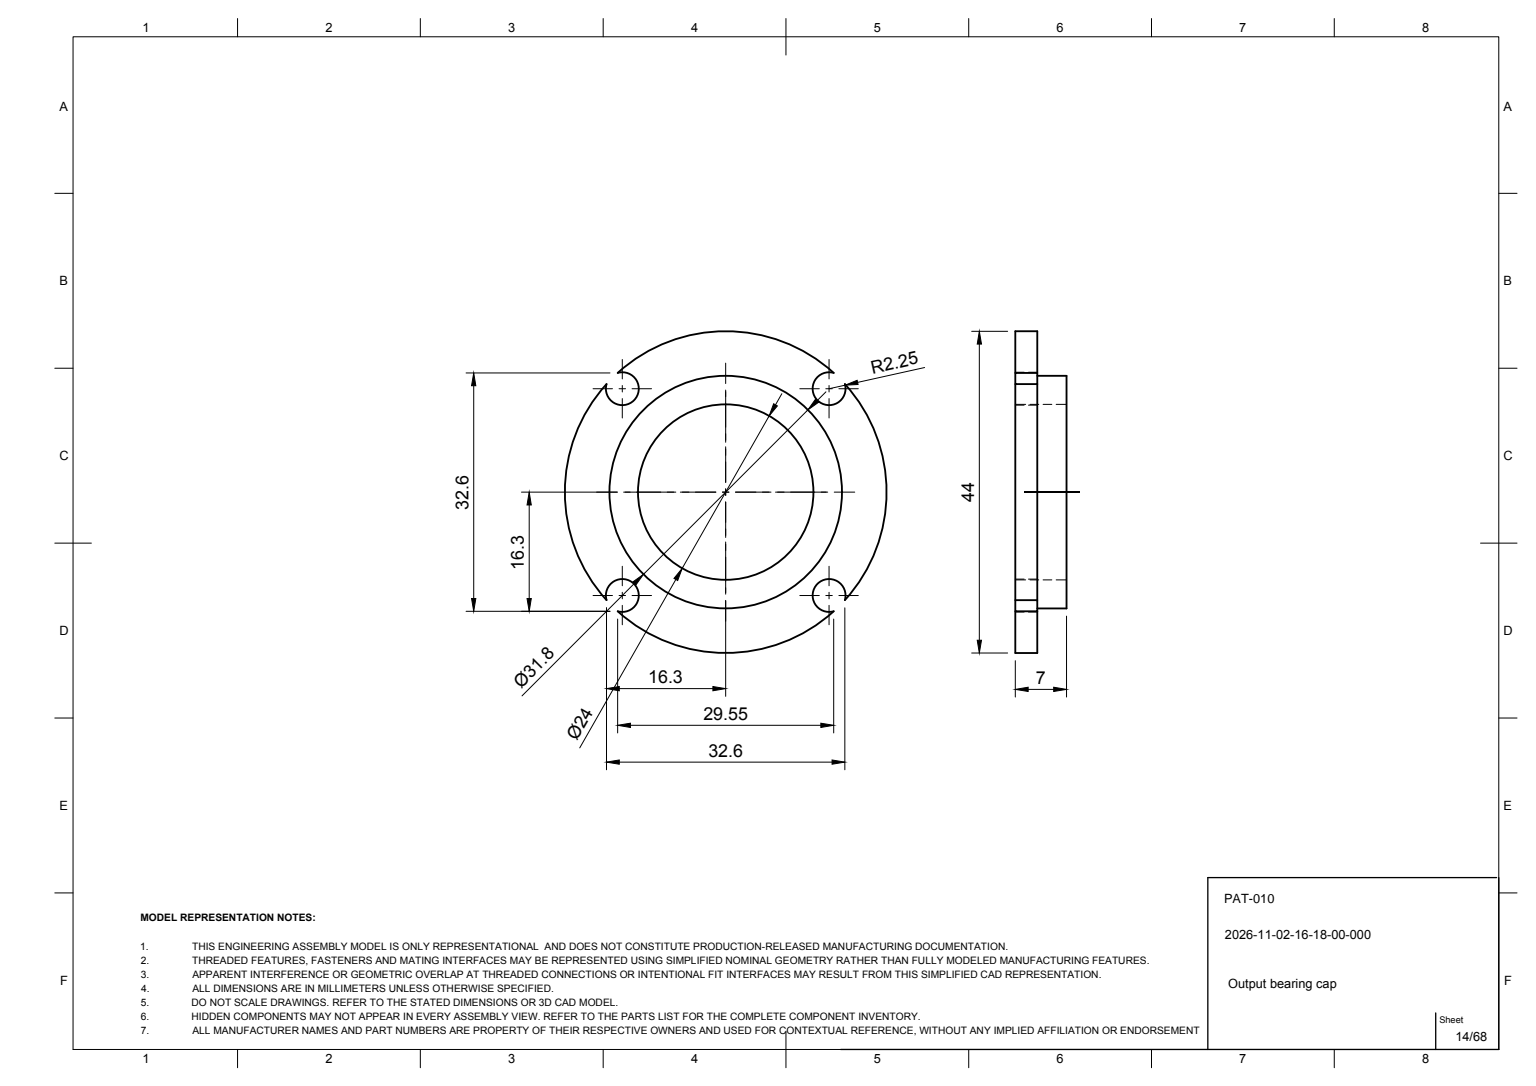
ISO-10303-21;
HEADER;
/* Generated by software containing ST-Developer
 * from STEP Tools, Inc. (www.steptools.com) 
 */

FILE_DESCRIPTION(
/* description */ ('Belt conveyor head drive unit'),
/* implementation_level */ '2;1');

FILE_NAME(
/* name */ 'Output bearing cap.step',
/* time_stamp */ '2026-10-28T03:26:19-07:00',
/* author */ (''),
/* organization */ (''),
/* preprocessor_version */ 'ST-DEVELOPER v20.2',
/* originating_system */ 'Autodesk Translation Framework v15.17.0.0',
/* authorisation */ '');

FILE_SCHEMA (('AUTOMOTIVE_DESIGN { 1 0 10303 214 3 1 1 }'));
ENDSEC;

DATA;
#10=MECHANICAL_DESIGN_GEOMETRIC_PRESENTATION_REPRESENTATION('',(#860),#27069);
#722=SHAPE_REPRESENTATION_RELATIONSHIP('SRR','None',#27366,#791);
#791=ADVANCED_BREP_SHAPE_REPRESENTATION('',(#945),#27008);
#860=STYLED_ITEM('',(#27797),#945);
#945=MANIFOLD_SOLID_BREP('Body1',#13725);
#1086=FACE_BOUND('',#2668,.T.);
#1087=FACE_BOUND('',#2675,.T.);
#1088=FACE_BOUND('',#2678,.T.);
#1358=PLANE('',#14900);
#1359=PLANE('',#14917);
#1360=PLANE('',#14920);
#1789=FACE_OUTER_BOUND('',#2663,.T.);
#1790=FACE_OUTER_BOUND('',#2664,.T.);
#1791=FACE_OUTER_BOUND('',#2665,.T.);
#1792=FACE_OUTER_BOUND('',#2666,.T.);
#1793=FACE_OUTER_BOUND('',#2667,.T.);
#1794=FACE_OUTER_BOUND('',#2669,.T.);
#1795=FACE_OUTER_BOUND('',#2670,.T.);
#1796=FACE_OUTER_BOUND('',#2671,.T.);
#1797=FACE_OUTER_BOUND('',#2672,.T.);
#1798=FACE_OUTER_BOUND('',#2673,.T.);
#1799=FACE_OUTER_BOUND('',#2674,.T.);
#1800=FACE_OUTER_BOUND('',#2676,.T.);
#1801=FACE_OUTER_BOUND('',#2677,.T.);
#2663=EDGE_LOOP('',(#9654,#9655,#9656,#9657));
#2664=EDGE_LOOP('',(#9658,#9659,#9660,#9661));
#2665=EDGE_LOOP('',(#9662,#9663,#9664,#9665));
#2666=EDGE_LOOP('',(#9666,#9667,#9668,#9669));
#2667=EDGE_LOOP('',(#9670,#9671,#9672,#9673,#9674,#9675,#9676,#9677));
#2668=EDGE_LOOP('',(#9678));
#2669=EDGE_LOOP('',(#9679,#9680,#9681,#9682));
#2670=EDGE_LOOP('',(#9683,#9684,#9685,#9686));
#2671=EDGE_LOOP('',(#9687,#9688,#9689,#9690));
#2672=EDGE_LOOP('',(#9691,#9692,#9693,#9694));
#2673=EDGE_LOOP('',(#9695,#9696,#9697,#9698));
#2674=EDGE_LOOP('',(#9699));
#2675=EDGE_LOOP('',(#9700));
#2676=EDGE_LOOP('',(#9701,#9702,#9703,#9704));
#2677=EDGE_LOOP('',(#9705,#9706,#9707,#9708,#9709,#9710,#9711,#9712));
#2678=EDGE_LOOP('',(#9713));
#3692=LINE('',#21725,#4484);
#3693=LINE('',#21729,#4485);
#3694=LINE('',#21734,#4486);
#3695=LINE('',#21738,#4487);
#3696=LINE('',#21743,#4488);
#3697=LINE('',#21747,#4489);
#3698=LINE('',#21752,#4490);
#3699=LINE('',#21756,#4491);
#3700=LINE('',#21777,#4492);
#3701=LINE('',#21783,#4493);
#4484=VECTOR('',#17282,1.);
#4485=VECTOR('',#17285,1.);
#4486=VECTOR('',#17290,1.);
#4487=VECTOR('',#17293,1.);
#4488=VECTOR('',#17298,1.);
#4489=VECTOR('',#17301,1.);
#4490=VECTOR('',#17306,1.);
#4491=VECTOR('',#17309,1.);
#4492=VECTOR('',#17344,1.59);
#4493=VECTOR('',#17353,1.2);
#5236=CIRCLE('',#14889,0.225);
#5237=CIRCLE('',#14890,0.225);
#5238=CIRCLE('',#14892,0.225);
#5239=CIRCLE('',#14893,0.225);
#5240=CIRCLE('',#14895,0.225);
#5241=CIRCLE('',#14896,0.225);
#5242=CIRCLE('',#14898,0.225);
#5243=CIRCLE('',#14899,0.225);
#5244=CIRCLE('',#14901,2.2);
#5245=CIRCLE('',#14902,2.2);
#5246=CIRCLE('',#14903,2.2);
#5247=CIRCLE('',#14904,2.2);
#5248=CIRCLE('',#14905,1.2);
#5249=CIRCLE('',#14907,2.2);
#5250=CIRCLE('',#14909,2.2);
#5251=CIRCLE('',#14911,2.2);
#5252=CIRCLE('',#14913,2.2);
#5253=CIRCLE('',#14915,1.59);
#5254=CIRCLE('',#14916,1.59);
#5255=CIRCLE('',#14918,1.2);
#6185=VERTEX_POINT('',#21723);
#6186=VERTEX_POINT('',#21724);
#6187=VERTEX_POINT('',#21726);
#6188=VERTEX_POINT('',#21728);
#6189=VERTEX_POINT('',#21732);
#6190=VERTEX_POINT('',#21733);
#6191=VERTEX_POINT('',#21735);
#6192=VERTEX_POINT('',#21737);
#6193=VERTEX_POINT('',#21741);
#6194=VERTEX_POINT('',#21742);
#6195=VERTEX_POINT('',#21744);
#6196=VERTEX_POINT('',#21746);
#6197=VERTEX_POINT('',#21750);
#6198=VERTEX_POINT('',#21751);
#6199=VERTEX_POINT('',#21753);
#6200=VERTEX_POINT('',#21755);
#6201=VERTEX_POINT('',#21763);
#6202=VERTEX_POINT('',#21774);
#6203=VERTEX_POINT('',#21776);
#6204=VERTEX_POINT('',#21780);
#7519=EDGE_CURVE('',#6185,#6186,#3692,.T.);
#7520=EDGE_CURVE('',#6187,#6185,#5236,.T.);
#7521=EDGE_CURVE('',#6188,#6187,#3693,.T.);
#7522=EDGE_CURVE('',#6186,#6188,#5237,.T.);
#7523=EDGE_CURVE('',#6189,#6190,#3694,.T.);
#7524=EDGE_CURVE('',#6191,#6189,#5238,.T.);
#7525=EDGE_CURVE('',#6192,#6191,#3695,.T.);
#7526=EDGE_CURVE('',#6190,#6192,#5239,.T.);
#7527=EDGE_CURVE('',#6193,#6194,#3696,.T.);
#7528=EDGE_CURVE('',#6195,#6193,#5240,.T.);
#7529=EDGE_CURVE('',#6196,#6195,#3697,.T.);
#7530=EDGE_CURVE('',#6194,#6196,#5241,.T.);
#7531=EDGE_CURVE('',#6197,#6198,#3698,.T.);
#7532=EDGE_CURVE('',#6199,#6197,#5242,.T.);
#7533=EDGE_CURVE('',#6200,#6199,#3699,.T.);
#7534=EDGE_CURVE('',#6198,#6200,#5243,.T.);
#7535=EDGE_CURVE('',#6199,#6185,#5244,.T.);
#7536=EDGE_CURVE('',#6195,#6197,#5245,.T.);
#7537=EDGE_CURVE('',#6191,#6193,#5246,.T.);
#7538=EDGE_CURVE('',#6187,#6189,#5247,.T.);
#7539=EDGE_CURVE('',#6201,#6201,#5248,.T.);
#7540=EDGE_CURVE('',#6196,#6198,#5249,.T.);
#7541=EDGE_CURVE('',#6192,#6194,#5250,.T.);
#7542=EDGE_CURVE('',#6200,#6186,#5251,.T.);
#7543=EDGE_CURVE('',#6188,#6190,#5252,.T.);
#7544=EDGE_CURVE('',#6202,#6202,#5253,.T.);
#7545=EDGE_CURVE('',#6202,#6203,#3700,.T.);
#7546=EDGE_CURVE('',#6203,#6203,#5254,.T.);
#7547=EDGE_CURVE('',#6204,#6204,#5255,.T.);
#7548=EDGE_CURVE('',#6204,#6201,#3701,.T.);
#9654=ORIENTED_EDGE('',*,*,#7519,.F.);
#9655=ORIENTED_EDGE('',*,*,#7520,.F.);
#9656=ORIENTED_EDGE('',*,*,#7521,.F.);
#9657=ORIENTED_EDGE('',*,*,#7522,.F.);
#9658=ORIENTED_EDGE('',*,*,#7523,.F.);
#9659=ORIENTED_EDGE('',*,*,#7524,.F.);
#9660=ORIENTED_EDGE('',*,*,#7525,.F.);
#9661=ORIENTED_EDGE('',*,*,#7526,.F.);
#9662=ORIENTED_EDGE('',*,*,#7527,.F.);
#9663=ORIENTED_EDGE('',*,*,#7528,.F.);
#9664=ORIENTED_EDGE('',*,*,#7529,.F.);
#9665=ORIENTED_EDGE('',*,*,#7530,.F.);
#9666=ORIENTED_EDGE('',*,*,#7531,.F.);
#9667=ORIENTED_EDGE('',*,*,#7532,.F.);
#9668=ORIENTED_EDGE('',*,*,#7533,.F.);
#9669=ORIENTED_EDGE('',*,*,#7534,.F.);
#9670=ORIENTED_EDGE('',*,*,#7520,.T.);
#9671=ORIENTED_EDGE('',*,*,#7535,.F.);
#9672=ORIENTED_EDGE('',*,*,#7532,.T.);
#9673=ORIENTED_EDGE('',*,*,#7536,.F.);
#9674=ORIENTED_EDGE('',*,*,#7528,.T.);
#9675=ORIENTED_EDGE('',*,*,#7537,.F.);
#9676=ORIENTED_EDGE('',*,*,#7524,.T.);
#9677=ORIENTED_EDGE('',*,*,#7538,.F.);
#9678=ORIENTED_EDGE('',*,*,#7539,.F.);
#9679=ORIENTED_EDGE('',*,*,#7529,.T.);
#9680=ORIENTED_EDGE('',*,*,#7536,.T.);
#9681=ORIENTED_EDGE('',*,*,#7531,.T.);
#9682=ORIENTED_EDGE('',*,*,#7540,.F.);
#9683=ORIENTED_EDGE('',*,*,#7525,.T.);
#9684=ORIENTED_EDGE('',*,*,#7537,.T.);
#9685=ORIENTED_EDGE('',*,*,#7527,.T.);
#9686=ORIENTED_EDGE('',*,*,#7541,.F.);
#9687=ORIENTED_EDGE('',*,*,#7519,.T.);
#9688=ORIENTED_EDGE('',*,*,#7542,.F.);
#9689=ORIENTED_EDGE('',*,*,#7533,.T.);
#9690=ORIENTED_EDGE('',*,*,#7535,.T.);
#9691=ORIENTED_EDGE('',*,*,#7521,.T.);
#9692=ORIENTED_EDGE('',*,*,#7538,.T.);
#9693=ORIENTED_EDGE('',*,*,#7523,.T.);
#9694=ORIENTED_EDGE('',*,*,#7543,.F.);
#9695=ORIENTED_EDGE('',*,*,#7544,.F.);
#9696=ORIENTED_EDGE('',*,*,#7545,.T.);
#9697=ORIENTED_EDGE('',*,*,#7546,.F.);
#9698=ORIENTED_EDGE('',*,*,#7545,.F.);
#9699=ORIENTED_EDGE('',*,*,#7544,.T.);
#9700=ORIENTED_EDGE('',*,*,#7547,.T.);
#9701=ORIENTED_EDGE('',*,*,#7547,.F.);
#9702=ORIENTED_EDGE('',*,*,#7548,.T.);
#9703=ORIENTED_EDGE('',*,*,#7539,.T.);
#9704=ORIENTED_EDGE('',*,*,#7548,.F.);
#9705=ORIENTED_EDGE('',*,*,#7522,.T.);
#9706=ORIENTED_EDGE('',*,*,#7543,.T.);
#9707=ORIENTED_EDGE('',*,*,#7526,.T.);
#9708=ORIENTED_EDGE('',*,*,#7541,.T.);
#9709=ORIENTED_EDGE('',*,*,#7530,.T.);
#9710=ORIENTED_EDGE('',*,*,#7540,.T.);
#9711=ORIENTED_EDGE('',*,*,#7534,.T.);
#9712=ORIENTED_EDGE('',*,*,#7542,.T.);
#9713=ORIENTED_EDGE('',*,*,#7546,.T.);
#12607=CYLINDRICAL_SURFACE('',#14888,0.225);
#12608=CYLINDRICAL_SURFACE('',#14891,0.225);
#12609=CYLINDRICAL_SURFACE('',#14894,0.225);
#12610=CYLINDRICAL_SURFACE('',#14897,0.225);
#12611=CYLINDRICAL_SURFACE('',#14906,2.2);
#12612=CYLINDRICAL_SURFACE('',#14908,2.2);
#12613=CYLINDRICAL_SURFACE('',#14910,2.2);
#12614=CYLINDRICAL_SURFACE('',#14912,2.2);
#12615=CYLINDRICAL_SURFACE('',#14914,1.59);
#12616=CYLINDRICAL_SURFACE('',#14919,1.2);
#13068=ADVANCED_FACE('',(#1789),#12607,.F.);
#13069=ADVANCED_FACE('',(#1790),#12608,.F.);
#13070=ADVANCED_FACE('',(#1791),#12609,.F.);
#13071=ADVANCED_FACE('',(#1792),#12610,.F.);
#13072=ADVANCED_FACE('',(#1793,#1086),#1358,.F.);
#13073=ADVANCED_FACE('',(#1794),#12611,.T.);
#13074=ADVANCED_FACE('',(#1795),#12612,.T.);
#13075=ADVANCED_FACE('',(#1796),#12613,.T.);
#13076=ADVANCED_FACE('',(#1797),#12614,.T.);
#13077=ADVANCED_FACE('',(#1798),#12615,.T.);
#13078=ADVANCED_FACE('',(#1799,#1087),#1359,.T.);
#13079=ADVANCED_FACE('',(#1800),#12616,.F.);
#13080=ADVANCED_FACE('',(#1801,#1088),#1360,.T.);
#13725=CLOSED_SHELL('',(#13068,#13069,#13070,#13071,#13072,#13073,#13074,
#13075,#13076,#13077,#13078,#13079,#13080));
#14887=AXIS2_PLACEMENT_3D('',#21721,#17278,#17279);
#14888=AXIS2_PLACEMENT_3D('',#21722,#17280,#17281);
#14889=AXIS2_PLACEMENT_3D('',#21727,#17283,#17284);
#14890=AXIS2_PLACEMENT_3D('',#21730,#17286,#17287);
#14891=AXIS2_PLACEMENT_3D('',#21731,#17288,#17289);
#14892=AXIS2_PLACEMENT_3D('',#21736,#17291,#17292);
#14893=AXIS2_PLACEMENT_3D('',#21739,#17294,#17295);
#14894=AXIS2_PLACEMENT_3D('',#21740,#17296,#17297);
#14895=AXIS2_PLACEMENT_3D('',#21745,#17299,#17300);
#14896=AXIS2_PLACEMENT_3D('',#21748,#17302,#17303);
#14897=AXIS2_PLACEMENT_3D('',#21749,#17304,#17305);
#14898=AXIS2_PLACEMENT_3D('',#21754,#17307,#17308);
#14899=AXIS2_PLACEMENT_3D('',#21757,#17310,#17311);
#14900=AXIS2_PLACEMENT_3D('',#21758,#17312,#17313);
#14901=AXIS2_PLACEMENT_3D('',#21759,#17314,#17315);
#14902=AXIS2_PLACEMENT_3D('',#21760,#17316,#17317);
#14903=AXIS2_PLACEMENT_3D('',#21761,#17318,#17319);
#14904=AXIS2_PLACEMENT_3D('',#21762,#17320,#17321);
#14905=AXIS2_PLACEMENT_3D('',#21764,#17322,#17323);
#14906=AXIS2_PLACEMENT_3D('',#21765,#17324,#17325);
#14907=AXIS2_PLACEMENT_3D('',#21766,#17326,#17327);
#14908=AXIS2_PLACEMENT_3D('',#21767,#17328,#17329);
#14909=AXIS2_PLACEMENT_3D('',#21768,#17330,#17331);
#14910=AXIS2_PLACEMENT_3D('',#21769,#17332,#17333);
#14911=AXIS2_PLACEMENT_3D('',#21770,#17334,#17335);
#14912=AXIS2_PLACEMENT_3D('',#21771,#17336,#17337);
#14913=AXIS2_PLACEMENT_3D('',#21772,#17338,#17339);
#14914=AXIS2_PLACEMENT_3D('',#21773,#17340,#17341);
#14915=AXIS2_PLACEMENT_3D('',#21775,#17342,#17343);
#14916=AXIS2_PLACEMENT_3D('',#21778,#17345,#17346);
#14917=AXIS2_PLACEMENT_3D('',#21779,#17347,#17348);
#14918=AXIS2_PLACEMENT_3D('',#21781,#17349,#17350);
#14919=AXIS2_PLACEMENT_3D('',#21782,#17351,#17352);
#14920=AXIS2_PLACEMENT_3D('',#21784,#17354,#17355);
#17278=DIRECTION('axis',(0.,0.,1.));
#17279=DIRECTION('refdir',(1.,0.,0.));
#17280=DIRECTION('center_axis',(0.,1.,0.));
#17281=DIRECTION('ref_axis',(0.707106781186546,0.,0.707106781186549));
#17282=DIRECTION('',(0.,1.,0.));
#17283=DIRECTION('center_axis',(0.,1.,0.));
#17284=DIRECTION('ref_axis',(1.,0.,0.));
#17285=DIRECTION('',(0.,-1.,0.));
#17286=DIRECTION('center_axis',(0.,-1.,0.));
#17287=DIRECTION('ref_axis',(1.,0.,0.));
#17288=DIRECTION('center_axis',(0.,1.,0.));
#17289=DIRECTION('ref_axis',(0.707106781186544,0.,-0.707106781186551));
#17290=DIRECTION('',(0.,1.,0.));
#17291=DIRECTION('center_axis',(0.,1.,0.));
#17292=DIRECTION('ref_axis',(1.,0.,0.));
#17293=DIRECTION('',(0.,-1.,0.));
#17294=DIRECTION('center_axis',(0.,-1.,0.));
#17295=DIRECTION('ref_axis',(1.,0.,0.));
#17296=DIRECTION('center_axis',(0.,1.,0.));
#17297=DIRECTION('ref_axis',(-0.707106781186548,0.,-0.707106781186547));
#17298=DIRECTION('',(0.,1.,0.));
#17299=DIRECTION('center_axis',(0.,1.,0.));
#17300=DIRECTION('ref_axis',(1.,0.,0.));
#17301=DIRECTION('',(0.,-1.,0.));
#17302=DIRECTION('center_axis',(0.,-1.,0.));
#17303=DIRECTION('ref_axis',(1.,0.,0.));
#17304=DIRECTION('center_axis',(0.,1.,0.));
#17305=DIRECTION('ref_axis',(-0.707106781186544,0.,0.707106781186551));
#17306=DIRECTION('',(0.,1.,0.));
#17307=DIRECTION('center_axis',(0.,1.,0.));
#17308=DIRECTION('ref_axis',(1.,0.,0.));
#17309=DIRECTION('',(0.,-1.,0.));
#17310=DIRECTION('center_axis',(0.,-1.,0.));
#17311=DIRECTION('ref_axis',(1.,0.,0.));
#17312=DIRECTION('center_axis',(0.,1.,0.));
#17313=DIRECTION('ref_axis',(1.,0.,0.));
#17314=DIRECTION('center_axis',(0.,1.,0.));
#17315=DIRECTION('ref_axis',(1.,0.,0.));
#17316=DIRECTION('center_axis',(0.,1.,0.));
#17317=DIRECTION('ref_axis',(1.,0.,0.));
#17318=DIRECTION('center_axis',(0.,1.,0.));
#17319=DIRECTION('ref_axis',(1.,0.,0.));
#17320=DIRECTION('center_axis',(0.,1.,0.));
#17321=DIRECTION('ref_axis',(1.,0.,0.));
#17322=DIRECTION('center_axis',(0.,-1.,0.));
#17323=DIRECTION('ref_axis',(1.,0.,0.));
#17324=DIRECTION('center_axis',(0.,1.,0.));
#17325=DIRECTION('ref_axis',(1.,0.,0.));
#17326=DIRECTION('center_axis',(0.,1.,0.));
#17327=DIRECTION('ref_axis',(1.,0.,0.));
#17328=DIRECTION('center_axis',(0.,1.,0.));
#17329=DIRECTION('ref_axis',(1.,0.,0.));
#17330=DIRECTION('center_axis',(0.,1.,0.));
#17331=DIRECTION('ref_axis',(1.,0.,0.));
#17332=DIRECTION('center_axis',(0.,1.,0.));
#17333=DIRECTION('ref_axis',(1.,0.,0.));
#17334=DIRECTION('center_axis',(0.,1.,0.));
#17335=DIRECTION('ref_axis',(1.,0.,0.));
#17336=DIRECTION('center_axis',(0.,1.,0.));
#17337=DIRECTION('ref_axis',(-1.,0.,-1.01064309961486E-15));
#17338=DIRECTION('center_axis',(0.,1.,0.));
#17339=DIRECTION('ref_axis',(1.,0.,0.));
#17340=DIRECTION('center_axis',(0.,1.,0.));
#17341=DIRECTION('ref_axis',(1.,0.,0.));
#17342=DIRECTION('center_axis',(0.,1.,0.));
#17343=DIRECTION('ref_axis',(1.,0.,0.));
#17344=DIRECTION('',(0.,-1.,0.));
#17345=DIRECTION('center_axis',(0.,-1.,0.));
#17346=DIRECTION('ref_axis',(1.,0.,0.));
#17347=DIRECTION('center_axis',(0.,1.,0.));
#17348=DIRECTION('ref_axis',(1.,0.,0.));
#17349=DIRECTION('center_axis',(0.,-1.,0.));
#17350=DIRECTION('ref_axis',(1.,0.,0.));
#17351=DIRECTION('center_axis',(0.,1.,0.));
#17352=DIRECTION('ref_axis',(1.,0.,0.));
#17353=DIRECTION('',(0.,-1.,0.));
#17354=DIRECTION('center_axis',(0.,1.,0.));
#17355=DIRECTION('ref_axis',(1.,0.,0.));
#21721=CARTESIAN_POINT('',(0.,0.,0.));
#21722=CARTESIAN_POINT('Origin',(5.55669646780806,-2.2,5.58578643762691));
#21723=CARTESIAN_POINT('',(5.49357471024299,-2.1,5.36982198749241));
#21724=CARTESIAN_POINT('',(5.49357471024299,-1.8,5.36982198749241));
#21725=CARTESIAN_POINT('',(5.49357471024299,-2.2,5.36982198749241));
#21726=CARTESIAN_POINT('',(5.34073201767356,-2.1,5.52266468006184));
#21727=CARTESIAN_POINT('Origin',(5.55669646780806,-2.1,5.58578643762691));
#21728=CARTESIAN_POINT('',(5.34073201767356,-1.8,5.52266468006184));
#21729=CARTESIAN_POINT('',(5.34073201767356,-2.2,5.52266468006184));
#21730=CARTESIAN_POINT('Origin',(5.55669646780806,-1.8,5.58578643762691));
#21731=CARTESIAN_POINT('Origin',(5.55669646780806,-2.2,8.4142135623731));
#21732=CARTESIAN_POINT('',(5.34073201767356,-2.1,8.47733531993816));
#21733=CARTESIAN_POINT('',(5.34073201767356,-1.8,8.47733531993816));
#21734=CARTESIAN_POINT('',(5.34073201767356,-2.2,8.47733531993816));
#21735=CARTESIAN_POINT('',(5.493574710243,-2.1,8.6301780125076));
#21736=CARTESIAN_POINT('Origin',(5.55669646780806,-2.1,8.4142135623731));
#21737=CARTESIAN_POINT('',(5.493574710243,-1.8,8.6301780125076));
#21738=CARTESIAN_POINT('',(5.493574710243,-2.2,8.6301780125076));
#21739=CARTESIAN_POINT('Origin',(5.55669646780806,-1.8,8.4142135623731));
#21740=CARTESIAN_POINT('Origin',(8.38512359255425,-2.2,8.4142135623731));
#21741=CARTESIAN_POINT('',(8.44824535011931,-2.1,8.6301780125076));
#21742=CARTESIAN_POINT('',(8.44824535011931,-1.8,8.6301780125076));
#21743=CARTESIAN_POINT('',(8.44824535011932,-2.2,8.6301780125076));
#21744=CARTESIAN_POINT('',(8.60108804268875,-2.1,8.47733531993816));
#21745=CARTESIAN_POINT('Origin',(8.38512359255425,-2.1,8.4142135623731));
#21746=CARTESIAN_POINT('',(8.60108804268875,-1.8,8.47733531993816));
#21747=CARTESIAN_POINT('',(8.60108804268875,-2.2,8.47733531993816));
#21748=CARTESIAN_POINT('Origin',(8.38512359255425,-1.8,8.4142135623731));
#21749=CARTESIAN_POINT('Origin',(8.38512359255425,-2.2,5.58578643762691));
#21750=CARTESIAN_POINT('',(8.60108804268875,-2.1,5.52266468006184));
#21751=CARTESIAN_POINT('',(8.60108804268875,-1.8,5.52266468006184));
#21752=CARTESIAN_POINT('',(8.60108804268875,-2.2,5.52266468006184));
#21753=CARTESIAN_POINT('',(8.44824535011932,-2.1,5.36982198749241));
#21754=CARTESIAN_POINT('Origin',(8.38512359255425,-2.1,5.58578643762691));
#21755=CARTESIAN_POINT('',(8.44824535011932,-1.8,5.36982198749241));
#21756=CARTESIAN_POINT('',(8.44824535011932,-2.2,5.36982198749241));
#21757=CARTESIAN_POINT('Origin',(8.38512359255425,-1.8,5.58578643762691));
#21758=CARTESIAN_POINT('Origin',(6.97091003018116,-2.1,7.));
#21759=CARTESIAN_POINT('Origin',(6.97091003018116,-2.1,7.));
#21760=CARTESIAN_POINT('Origin',(6.97091003018116,-2.1,7.));
#21761=CARTESIAN_POINT('Origin',(6.97091003018116,-2.1,7.));
#21762=CARTESIAN_POINT('Origin',(6.97091003018116,-2.1,7.));
#21763=CARTESIAN_POINT('',(5.77091003018116,-2.1,7.));
#21764=CARTESIAN_POINT('Origin',(6.97091003018116,-2.1,7.));
#21765=CARTESIAN_POINT('Origin',(6.97091003018116,-2.1,7.));
#21766=CARTESIAN_POINT('Origin',(6.97091003018116,-1.8,7.));
#21767=CARTESIAN_POINT('Origin',(6.97091003018116,-2.1,7.));
#21768=CARTESIAN_POINT('Origin',(6.97091003018116,-1.8,7.));
#21769=CARTESIAN_POINT('Origin',(6.97091003018116,-2.1,7.));
#21770=CARTESIAN_POINT('Origin',(6.97091003018116,-1.8,7.));
#21771=CARTESIAN_POINT('Origin',(6.97091003018116,-2.1,7.));
#21772=CARTESIAN_POINT('Origin',(6.97091003018116,-1.8,7.));
#21773=CARTESIAN_POINT('Origin',(6.97091003018116,-1.8,7.));
#21774=CARTESIAN_POINT('',(5.38091003018116,-1.4,7.));
#21775=CARTESIAN_POINT('Origin',(6.97091003018116,-1.4,7.));
#21776=CARTESIAN_POINT('',(5.38091003018116,-1.8,7.));
#21777=CARTESIAN_POINT('',(5.38091003018116,-1.8,7.));
#21778=CARTESIAN_POINT('Origin',(6.97091003018116,-1.8,7.));
#21779=CARTESIAN_POINT('Origin',(6.97091003018116,-1.4,7.));
#21780=CARTESIAN_POINT('',(5.77091003018116,-1.4,7.));
#21781=CARTESIAN_POINT('Origin',(6.97091003018116,-1.4,7.));
#21782=CARTESIAN_POINT('Origin',(6.97091003018116,-2.1,7.));
#21783=CARTESIAN_POINT('',(5.77091003018116,-2.1,7.));
#21784=CARTESIAN_POINT('Origin',(6.97091003018116,-1.8,7.));
#26931=UNCERTAINTY_MEASURE_WITH_UNIT(LENGTH_MEASURE(0.001),#27070,
'DISTANCE_ACCURACY_VALUE',
'Maximum model space distance between geometric entities at asserted c
onnectivities');
#26992=UNCERTAINTY_MEASURE_WITH_UNIT(LENGTH_MEASURE(0.001),#27070,
'DISTANCE_ACCURACY_VALUE',
'Maximum model space distance between geometric entities at asserted c
onnectivities');
#27008=(
GEOMETRIC_REPRESENTATION_CONTEXT(3)
GLOBAL_UNCERTAINTY_ASSIGNED_CONTEXT((#26931))
GLOBAL_UNIT_ASSIGNED_CONTEXT((#27070,#27072,#27073))
REPRESENTATION_CONTEXT('','3D')
);
#27069=(
GEOMETRIC_REPRESENTATION_CONTEXT(3)
GLOBAL_UNCERTAINTY_ASSIGNED_CONTEXT((#26992))
GLOBAL_UNIT_ASSIGNED_CONTEXT((#27070,#27072,#27073))
REPRESENTATION_CONTEXT('','3D')
);
#27070=(
LENGTH_UNIT()
NAMED_UNIT(*)
SI_UNIT(.CENTI.,.METRE.)
);
#27072=(
NAMED_UNIT(*)
PLANE_ANGLE_UNIT()
SI_UNIT($,.RADIAN.)
);
#27073=(
NAMED_UNIT(*)
SI_UNIT($,.STERADIAN.)
SOLID_ANGLE_UNIT()
);
#27089=SHAPE_DEFINITION_REPRESENTATION(#27165,#27366);
#27165=PRODUCT_DEFINITION_SHAPE('',$,#27443);
#27366=SHAPE_REPRESENTATION('',(#14887),#27008);
#27427=PRODUCT_DEFINITION_CONTEXT('part definition',#27657,'design');
#27443=PRODUCT_DEFINITION('Output bearing cap','Output bearing cap',#27519,
#27427);
#27519=PRODUCT_DEFINITION_FORMATION('',$,#27674);
#27657=APPLICATION_CONTEXT(
'Core Data for Automotive Mechanical Design Process');
#27658=PRODUCT_CONTEXT('part definition',#27657,'mechanical');
#27674=PRODUCT('Output bearing cap','Output bearing cap',
'Output bearing cap',(#27658));
#27791=COLOUR_RGB('Grey',0.48,0.52,0.57);
#27792=FILL_AREA_STYLE_COLOUR('',#27791);
#27793=FILL_AREA_STYLE('',(#27792));
#27794=SURFACE_STYLE_FILL_AREA(#27793);
#27795=SURFACE_SIDE_STYLE('',(#27794));
#27796=SURFACE_STYLE_USAGE(.BOTH.,#27795);
#27797=PRESENTATION_STYLE_ASSIGNMENT((#27796));
ENDSEC;
END-ISO-10303-21;
